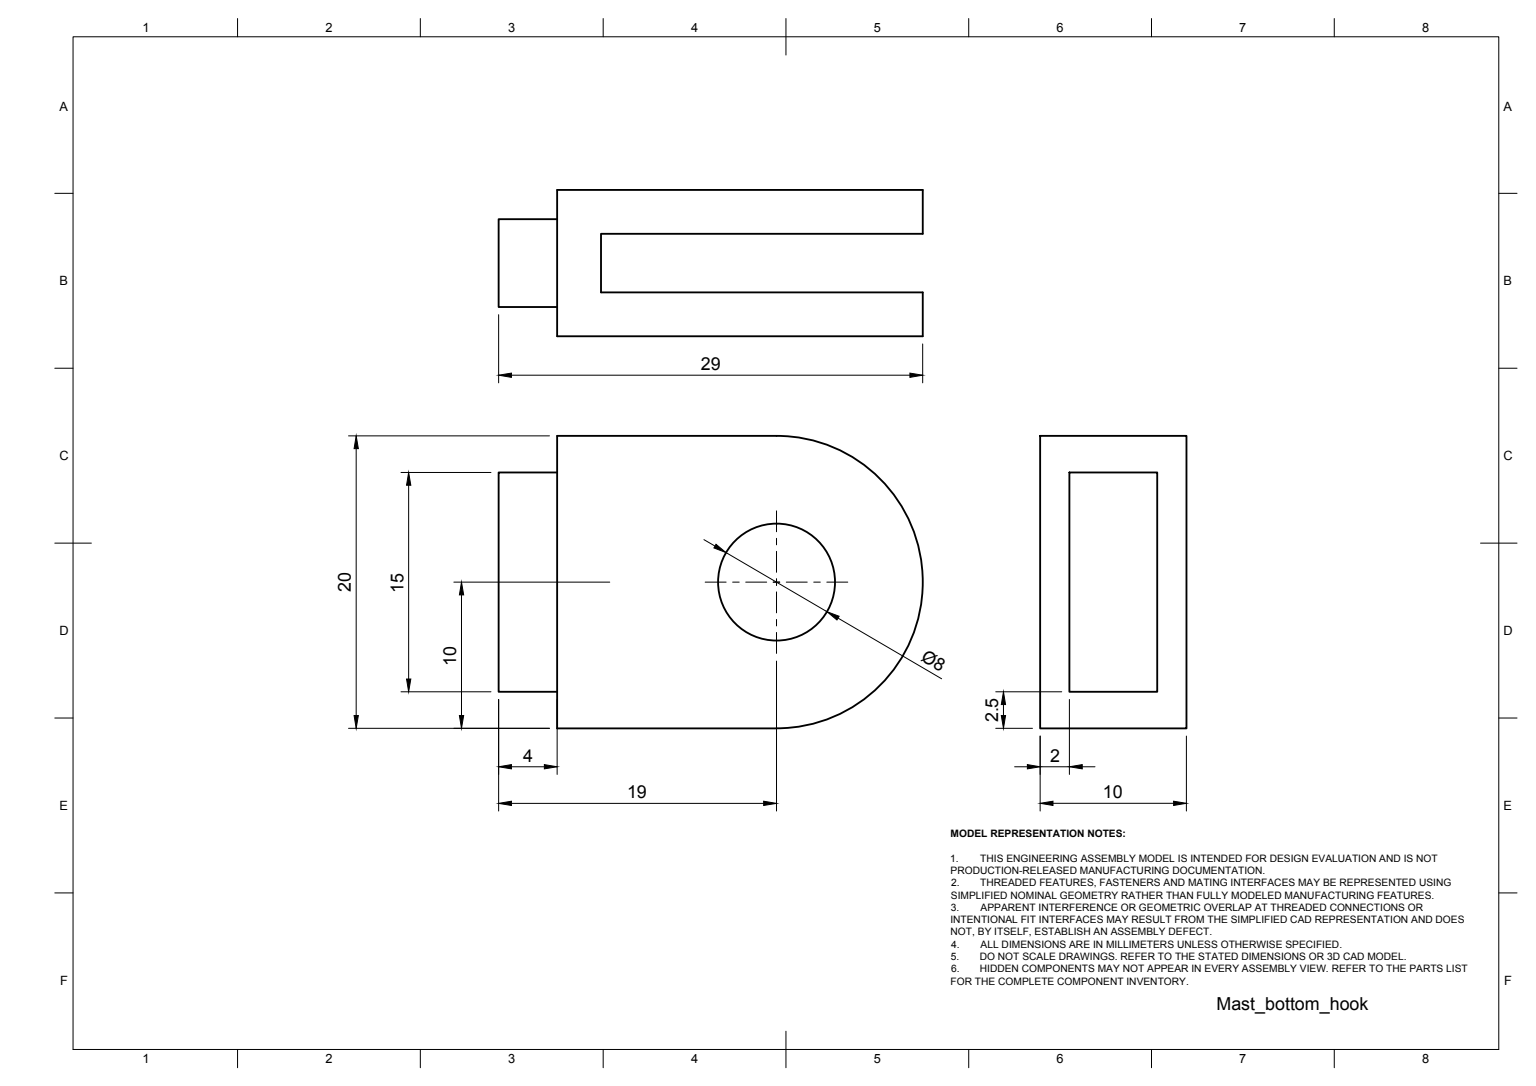
ISO-10303-21;
HEADER;
/* Generated by software containing ST-Developer
 * from STEP Tools, Inc. (www.steptools.com) 
 */

FILE_DESCRIPTION(
/* description */ (''),
/* implementation_level */ '2;1');

FILE_NAME(
/* name */ 'Mast_bottom_hook.step',
/* time_stamp */ '2026-10-07T11:02:43-07:00',
/* author */ (''),
/* organization */ (''),
/* preprocessor_version */ 'ST-DEVELOPER v20.2',
/* originating_system */ 'Autodesk Translation Framework v15.15.0.0',
/* authorisation */ '');

FILE_SCHEMA (('AUTOMOTIVE_DESIGN { 1 0 10303 214 3 1 1 }'));
ENDSEC;

DATA;
#10=MECHANICAL_DESIGN_GEOMETRIC_PRESENTATION_REPRESENTATION('',(#71),#5505);
#57=SHAPE_REPRESENTATION_RELATIONSHIP('SRR','None',#5542,#64);
#64=ADVANCED_BREP_SHAPE_REPRESENTATION('',(#78),#5503);
#71=STYLED_ITEM('',(#5586),#78);
#78=MANIFOLD_SOLID_BREP('Body1',#3298);
#103=FACE_BOUND('',#554,.T.);
#104=FACE_BOUND('',#556,.T.);
#105=FACE_BOUND('',#558,.T.);
#106=FACE_BOUND('',#560,.T.);
#107=FACE_BOUND('',#562,.T.);
#143=CYLINDRICAL_SURFACE('',#3592,4.);
#144=CYLINDRICAL_SURFACE('',#3593,4.);
#145=CYLINDRICAL_SURFACE('',#3594,10.);
#146=CYLINDRICAL_SURFACE('',#3595,10.);
#216=CIRCLE('',#3578,10.);
#217=CIRCLE('',#3579,4.);
#218=CIRCLE('',#3581,10.);
#219=CIRCLE('',#3582,4.);
#220=CIRCLE('',#3584,10.);
#221=CIRCLE('',#3585,4.);
#222=CIRCLE('',#3587,10.);
#223=CIRCLE('',#3588,4.);
#364=FACE_OUTER_BOUND('',#553,.T.);
#365=FACE_OUTER_BOUND('',#555,.T.);
#366=FACE_OUTER_BOUND('',#557,.T.);
#367=FACE_OUTER_BOUND('',#559,.T.);
#368=FACE_OUTER_BOUND('',#561,.T.);
#369=FACE_OUTER_BOUND('',#563,.T.);
#370=FACE_OUTER_BOUND('',#564,.T.);
#371=FACE_OUTER_BOUND('',#565,.T.);
#372=FACE_OUTER_BOUND('',#566,.T.);
#373=FACE_OUTER_BOUND('',#567,.T.);
#374=FACE_OUTER_BOUND('',#568,.T.);
#375=FACE_OUTER_BOUND('',#569,.T.);
#376=FACE_OUTER_BOUND('',#570,.T.);
#377=FACE_OUTER_BOUND('',#571,.T.);
#378=FACE_OUTER_BOUND('',#572,.T.);
#379=FACE_OUTER_BOUND('',#573,.T.);
#380=FACE_OUTER_BOUND('',#574,.T.);
#553=EDGE_LOOP('',(#2810,#2811,#2812,#2813));
#554=EDGE_LOOP('',(#2814,#2815,#2816,#2817));
#555=EDGE_LOOP('',(#2818,#2819,#2820,#2821));
#556=EDGE_LOOP('',(#2822));
#557=EDGE_LOOP('',(#2823,#2824,#2825,#2826));
#558=EDGE_LOOP('',(#2827));
#559=EDGE_LOOP('',(#2828,#2829,#2830,#2831));
#560=EDGE_LOOP('',(#2832));
#561=EDGE_LOOP('',(#2833,#2834,#2835,#2836));
#562=EDGE_LOOP('',(#2837));
#563=EDGE_LOOP('',(#2838,#2839,#2840,#2841,#2842,#2843,#2844,#2845));
#564=EDGE_LOOP('',(#2846,#2847,#2848,#2849,#2850,#2851,#2852,#2853));
#565=EDGE_LOOP('',(#2854,#2855,#2856,#2857));
#566=EDGE_LOOP('',(#2858,#2859,#2860,#2861));
#567=EDGE_LOOP('',(#2862,#2863,#2864,#2865));
#568=EDGE_LOOP('',(#2866,#2867,#2868,#2869));
#569=EDGE_LOOP('',(#2870,#2871,#2872,#2873));
#570=EDGE_LOOP('',(#2874,#2875,#2876,#2877));
#571=EDGE_LOOP('',(#2878,#2879,#2880,#2881));
#572=EDGE_LOOP('',(#2882,#2883,#2884,#2885));
#573=EDGE_LOOP('',(#2886,#2887,#2888,#2889));
#574=EDGE_LOOP('',(#2890,#2891,#2892,#2893));
#895=LINE('',#5282,#1265);
#896=LINE('',#5284,#1266);
#897=LINE('',#5286,#1267);
#898=LINE('',#5287,#1268);
#899=LINE('',#5290,#1269);
#900=LINE('',#5292,#1270);
#901=LINE('',#5294,#1271);
#902=LINE('',#5295,#1272);
#903=LINE('',#5298,#1273);
#904=LINE('',#5301,#1274);
#905=LINE('',#5308,#1275);
#906=LINE('',#5309,#1276);
#907=LINE('',#5315,#1277);
#908=LINE('',#5319,#1278);
#909=LINE('',#5320,#1279);
#910=LINE('',#5326,#1280);
#911=LINE('',#5330,#1281);
#912=LINE('',#5331,#1282);
#913=LINE('',#5335,#1283);
#914=LINE('',#5336,#1284);
#915=LINE('',#5337,#1285);
#916=LINE('',#5339,#1286);
#917=LINE('',#5340,#1287);
#918=LINE('',#5341,#1288);
#919=LINE('',#5344,#1289);
#920=LINE('',#5346,#1290);
#921=LINE('',#5351,#1291);
#922=LINE('',#5353,#1292);
#923=LINE('',#5354,#1293);
#924=LINE('',#5357,#1294);
#925=LINE('',#5358,#1295);
#926=LINE('',#5361,#1296);
#927=LINE('',#5362,#1297);
#928=LINE('',#5364,#1298);
#1265=VECTOR('',#4337,1000.);
#1266=VECTOR('',#4338,1000.);
#1267=VECTOR('',#4339,1000.);
#1268=VECTOR('',#4340,1000.);
#1269=VECTOR('',#4341,1000.);
#1270=VECTOR('',#4342,1000.);
#1271=VECTOR('',#4343,1000.);
#1272=VECTOR('',#4344,1000.);
#1273=VECTOR('',#4347,1000.);
#1274=VECTOR('',#4350,1000.);
#1275=VECTOR('',#4357,1000.);
#1276=VECTOR('',#4358,1000.);
#1277=VECTOR('',#4363,1000.);
#1278=VECTOR('',#4366,1000.);
#1279=VECTOR('',#4367,1000.);
#1280=VECTOR('',#4372,1000.);
#1281=VECTOR('',#4375,1000.);
#1282=VECTOR('',#4376,1000.);
#1283=VECTOR('',#4381,1000.);
#1284=VECTOR('',#4382,1000.);
#1285=VECTOR('',#4383,1000.);
#1286=VECTOR('',#4386,1000.);
#1287=VECTOR('',#4387,1000.);
#1288=VECTOR('',#4388,1000.);
#1289=VECTOR('',#4393,4.);
#1290=VECTOR('',#4396,4.);
#1291=VECTOR('',#4403,1000.);
#1292=VECTOR('',#4404,1000.);
#1293=VECTOR('',#4405,1000.);
#1294=VECTOR('',#4408,1000.);
#1295=VECTOR('',#4409,1000.);
#1296=VECTOR('',#4412,1000.);
#1297=VECTOR('',#4413,1000.);
#1298=VECTOR('',#4416,1000.);
#1579=VERTEX_POINT('',#5280);
#1580=VERTEX_POINT('',#5281);
#1581=VERTEX_POINT('',#5283);
#1582=VERTEX_POINT('',#5285);
#1583=VERTEX_POINT('',#5288);
#1584=VERTEX_POINT('',#5289);
#1585=VERTEX_POINT('',#5291);
#1586=VERTEX_POINT('',#5293);
#1587=VERTEX_POINT('',#5297);
#1588=VERTEX_POINT('',#5299);
#1589=VERTEX_POINT('',#5302);
#1590=VERTEX_POINT('',#5305);
#1591=VERTEX_POINT('',#5306);
#1592=VERTEX_POINT('',#5310);
#1593=VERTEX_POINT('',#5313);
#1594=VERTEX_POINT('',#5314);
#1595=VERTEX_POINT('',#5316);
#1596=VERTEX_POINT('',#5318);
#1597=VERTEX_POINT('',#5321);
#1598=VERTEX_POINT('',#5324);
#1599=VERTEX_POINT('',#5325);
#1600=VERTEX_POINT('',#5327);
#1601=VERTEX_POINT('',#5329);
#1602=VERTEX_POINT('',#5332);
#1603=VERTEX_POINT('',#5350);
#1604=VERTEX_POINT('',#5352);
#1605=VERTEX_POINT('',#5356);
#1606=VERTEX_POINT('',#5360);
#2000=EDGE_CURVE('',#1579,#1580,#895,.T.);
#2001=EDGE_CURVE('',#1581,#1580,#896,.T.);
#2002=EDGE_CURVE('',#1582,#1581,#897,.T.);
#2003=EDGE_CURVE('',#1582,#1579,#898,.T.);
#2004=EDGE_CURVE('',#1583,#1584,#899,.T.);
#2005=EDGE_CURVE('',#1583,#1585,#900,.T.);
#2006=EDGE_CURVE('',#1585,#1586,#901,.T.);
#2007=EDGE_CURVE('',#1584,#1586,#902,.T.);
#2008=EDGE_CURVE('',#1587,#1579,#903,.T.);
#2009=EDGE_CURVE('',#1587,#1588,#216,.T.);
#2010=EDGE_CURVE('',#1588,#1580,#904,.T.);
#2011=EDGE_CURVE('',#1589,#1589,#217,.T.);
#2012=EDGE_CURVE('',#1590,#1591,#218,.T.);
#2013=EDGE_CURVE('',#1590,#1582,#905,.T.);
#2014=EDGE_CURVE('',#1591,#1581,#906,.T.);
#2015=EDGE_CURVE('',#1592,#1592,#219,.T.);
#2016=EDGE_CURVE('',#1593,#1594,#907,.T.);
#2017=EDGE_CURVE('',#1594,#1595,#220,.T.);
#2018=EDGE_CURVE('',#1596,#1595,#908,.T.);
#2019=EDGE_CURVE('',#1596,#1593,#909,.T.);
#2020=EDGE_CURVE('',#1597,#1597,#221,.T.);
#2021=EDGE_CURVE('',#1598,#1599,#910,.T.);
#2022=EDGE_CURVE('',#1600,#1599,#222,.T.);
#2023=EDGE_CURVE('',#1601,#1600,#911,.T.);
#2024=EDGE_CURVE('',#1598,#1601,#912,.T.);
#2025=EDGE_CURVE('',#1602,#1602,#223,.T.);
#2026=EDGE_CURVE('',#1595,#1587,#913,.T.);
#2027=EDGE_CURVE('',#1590,#1599,#914,.T.);
#2028=EDGE_CURVE('',#1598,#1596,#915,.T.);
#2029=EDGE_CURVE('',#1594,#1588,#916,.T.);
#2030=EDGE_CURVE('',#1601,#1593,#917,.T.);
#2031=EDGE_CURVE('',#1591,#1600,#918,.T.);
#2032=EDGE_CURVE('',#1592,#1602,#919,.T.);
#2033=EDGE_CURVE('',#1597,#1589,#920,.T.);
#2034=EDGE_CURVE('',#1603,#1584,#921,.T.);
#2035=EDGE_CURVE('',#1604,#1603,#922,.T.);
#2036=EDGE_CURVE('',#1604,#1583,#923,.T.);
#2037=EDGE_CURVE('',#1604,#1605,#924,.T.);
#2038=EDGE_CURVE('',#1605,#1585,#925,.T.);
#2039=EDGE_CURVE('',#1605,#1606,#926,.T.);
#2040=EDGE_CURVE('',#1606,#1586,#927,.T.);
#2041=EDGE_CURVE('',#1603,#1606,#928,.T.);
#2810=ORIENTED_EDGE('',*,*,#2000,.T.);
#2811=ORIENTED_EDGE('',*,*,#2001,.F.);
#2812=ORIENTED_EDGE('',*,*,#2002,.F.);
#2813=ORIENTED_EDGE('',*,*,#2003,.T.);
#2814=ORIENTED_EDGE('',*,*,#2004,.F.);
#2815=ORIENTED_EDGE('',*,*,#2005,.T.);
#2816=ORIENTED_EDGE('',*,*,#2006,.T.);
#2817=ORIENTED_EDGE('',*,*,#2007,.F.);
#2818=ORIENTED_EDGE('',*,*,#2008,.F.);
#2819=ORIENTED_EDGE('',*,*,#2009,.T.);
#2820=ORIENTED_EDGE('',*,*,#2010,.T.);
#2821=ORIENTED_EDGE('',*,*,#2000,.F.);
#2822=ORIENTED_EDGE('',*,*,#2011,.F.);
#2823=ORIENTED_EDGE('',*,*,#2012,.F.);
#2824=ORIENTED_EDGE('',*,*,#2013,.T.);
#2825=ORIENTED_EDGE('',*,*,#2002,.T.);
#2826=ORIENTED_EDGE('',*,*,#2014,.F.);
#2827=ORIENTED_EDGE('',*,*,#2015,.T.);
#2828=ORIENTED_EDGE('',*,*,#2016,.T.);
#2829=ORIENTED_EDGE('',*,*,#2017,.T.);
#2830=ORIENTED_EDGE('',*,*,#2018,.F.);
#2831=ORIENTED_EDGE('',*,*,#2019,.T.);
#2832=ORIENTED_EDGE('',*,*,#2020,.F.);
#2833=ORIENTED_EDGE('',*,*,#2021,.T.);
#2834=ORIENTED_EDGE('',*,*,#2022,.F.);
#2835=ORIENTED_EDGE('',*,*,#2023,.F.);
#2836=ORIENTED_EDGE('',*,*,#2024,.F.);
#2837=ORIENTED_EDGE('',*,*,#2025,.T.);
#2838=ORIENTED_EDGE('',*,*,#2026,.T.);
#2839=ORIENTED_EDGE('',*,*,#2008,.T.);
#2840=ORIENTED_EDGE('',*,*,#2003,.F.);
#2841=ORIENTED_EDGE('',*,*,#2013,.F.);
#2842=ORIENTED_EDGE('',*,*,#2027,.T.);
#2843=ORIENTED_EDGE('',*,*,#2021,.F.);
#2844=ORIENTED_EDGE('',*,*,#2028,.T.);
#2845=ORIENTED_EDGE('',*,*,#2018,.T.);
#2846=ORIENTED_EDGE('',*,*,#2010,.F.);
#2847=ORIENTED_EDGE('',*,*,#2029,.F.);
#2848=ORIENTED_EDGE('',*,*,#2016,.F.);
#2849=ORIENTED_EDGE('',*,*,#2030,.F.);
#2850=ORIENTED_EDGE('',*,*,#2023,.T.);
#2851=ORIENTED_EDGE('',*,*,#2031,.F.);
#2852=ORIENTED_EDGE('',*,*,#2014,.T.);
#2853=ORIENTED_EDGE('',*,*,#2001,.T.);
#2854=ORIENTED_EDGE('',*,*,#2024,.T.);
#2855=ORIENTED_EDGE('',*,*,#2030,.T.);
#2856=ORIENTED_EDGE('',*,*,#2019,.F.);
#2857=ORIENTED_EDGE('',*,*,#2028,.F.);
#2858=ORIENTED_EDGE('',*,*,#2015,.F.);
#2859=ORIENTED_EDGE('',*,*,#2032,.T.);
#2860=ORIENTED_EDGE('',*,*,#2025,.F.);
#2861=ORIENTED_EDGE('',*,*,#2032,.F.);
#2862=ORIENTED_EDGE('',*,*,#2020,.T.);
#2863=ORIENTED_EDGE('',*,*,#2033,.T.);
#2864=ORIENTED_EDGE('',*,*,#2011,.T.);
#2865=ORIENTED_EDGE('',*,*,#2033,.F.);
#2866=ORIENTED_EDGE('',*,*,#2012,.T.);
#2867=ORIENTED_EDGE('',*,*,#2031,.T.);
#2868=ORIENTED_EDGE('',*,*,#2022,.T.);
#2869=ORIENTED_EDGE('',*,*,#2027,.F.);
#2870=ORIENTED_EDGE('',*,*,#2017,.F.);
#2871=ORIENTED_EDGE('',*,*,#2029,.T.);
#2872=ORIENTED_EDGE('',*,*,#2009,.F.);
#2873=ORIENTED_EDGE('',*,*,#2026,.F.);
#2874=ORIENTED_EDGE('',*,*,#2004,.T.);
#2875=ORIENTED_EDGE('',*,*,#2034,.F.);
#2876=ORIENTED_EDGE('',*,*,#2035,.F.);
#2877=ORIENTED_EDGE('',*,*,#2036,.T.);
#2878=ORIENTED_EDGE('',*,*,#2005,.F.);
#2879=ORIENTED_EDGE('',*,*,#2036,.F.);
#2880=ORIENTED_EDGE('',*,*,#2037,.T.);
#2881=ORIENTED_EDGE('',*,*,#2038,.T.);
#2882=ORIENTED_EDGE('',*,*,#2006,.F.);
#2883=ORIENTED_EDGE('',*,*,#2038,.F.);
#2884=ORIENTED_EDGE('',*,*,#2039,.T.);
#2885=ORIENTED_EDGE('',*,*,#2040,.T.);
#2886=ORIENTED_EDGE('',*,*,#2007,.T.);
#2887=ORIENTED_EDGE('',*,*,#2040,.F.);
#2888=ORIENTED_EDGE('',*,*,#2041,.F.);
#2889=ORIENTED_EDGE('',*,*,#2034,.T.);
#2890=ORIENTED_EDGE('',*,*,#2035,.T.);
#2891=ORIENTED_EDGE('',*,*,#2041,.T.);
#2892=ORIENTED_EDGE('',*,*,#2039,.F.);
#2893=ORIENTED_EDGE('',*,*,#2037,.F.);
#3099=PLANE('',#3576);
#3100=PLANE('',#3577);
#3101=PLANE('',#3580);
#3102=PLANE('',#3583);
#3103=PLANE('',#3586);
#3104=PLANE('',#3589);
#3105=PLANE('',#3590);
#3106=PLANE('',#3591);
#3107=PLANE('',#3596);
#3108=PLANE('',#3597);
#3109=PLANE('',#3598);
#3110=PLANE('',#3599);
#3111=PLANE('',#3600);
#3255=ADVANCED_FACE('',(#364,#103),#3099,.F.);
#3256=ADVANCED_FACE('',(#365,#104),#3100,.T.);
#3257=ADVANCED_FACE('',(#366,#105),#3101,.F.);
#3258=ADVANCED_FACE('',(#367,#106),#3102,.T.);
#3259=ADVANCED_FACE('',(#368,#107),#3103,.F.);
#3260=ADVANCED_FACE('',(#369),#3104,.T.);
#3261=ADVANCED_FACE('',(#370),#3105,.F.);
#3262=ADVANCED_FACE('',(#371),#3106,.T.);
#3263=ADVANCED_FACE('',(#372),#143,.F.);
#3264=ADVANCED_FACE('',(#373),#144,.F.);
#3265=ADVANCED_FACE('',(#374),#145,.T.);
#3266=ADVANCED_FACE('',(#375),#146,.T.);
#3267=ADVANCED_FACE('',(#376),#3107,.F.);
#3268=ADVANCED_FACE('',(#377),#3108,.T.);
#3269=ADVANCED_FACE('',(#378),#3109,.T.);
#3270=ADVANCED_FACE('',(#379),#3110,.F.);
#3271=ADVANCED_FACE('',(#380),#3111,.F.);
#3298=CLOSED_SHELL('',(#3255,#3256,#3257,#3258,#3259,#3260,#3261,#3262,
#3263,#3264,#3265,#3266,#3267,#3268,#3269,#3270,#3271));
#3575=AXIS2_PLACEMENT_3D('',#5278,#4333,#4334);
#3576=AXIS2_PLACEMENT_3D('',#5279,#4335,#4336);
#3577=AXIS2_PLACEMENT_3D('',#5296,#4345,#4346);
#3578=AXIS2_PLACEMENT_3D('',#5300,#4348,#4349);
#3579=AXIS2_PLACEMENT_3D('',#5303,#4351,#4352);
#3580=AXIS2_PLACEMENT_3D('',#5304,#4353,#4354);
#3581=AXIS2_PLACEMENT_3D('',#5307,#4355,#4356);
#3582=AXIS2_PLACEMENT_3D('',#5311,#4359,#4360);
#3583=AXIS2_PLACEMENT_3D('',#5312,#4361,#4362);
#3584=AXIS2_PLACEMENT_3D('',#5317,#4364,#4365);
#3585=AXIS2_PLACEMENT_3D('',#5322,#4368,#4369);
#3586=AXIS2_PLACEMENT_3D('',#5323,#4370,#4371);
#3587=AXIS2_PLACEMENT_3D('',#5328,#4373,#4374);
#3588=AXIS2_PLACEMENT_3D('',#5333,#4377,#4378);
#3589=AXIS2_PLACEMENT_3D('',#5334,#4379,#4380);
#3590=AXIS2_PLACEMENT_3D('',#5338,#4384,#4385);
#3591=AXIS2_PLACEMENT_3D('',#5342,#4389,#4390);
#3592=AXIS2_PLACEMENT_3D('',#5343,#4391,#4392);
#3593=AXIS2_PLACEMENT_3D('',#5345,#4394,#4395);
#3594=AXIS2_PLACEMENT_3D('',#5347,#4397,#4398);
#3595=AXIS2_PLACEMENT_3D('',#5348,#4399,#4400);
#3596=AXIS2_PLACEMENT_3D('',#5349,#4401,#4402);
#3597=AXIS2_PLACEMENT_3D('',#5355,#4406,#4407);
#3598=AXIS2_PLACEMENT_3D('',#5359,#4410,#4411);
#3599=AXIS2_PLACEMENT_3D('',#5363,#4414,#4415);
#3600=AXIS2_PLACEMENT_3D('',#5365,#4417,#4418);
#4333=DIRECTION('axis',(0.,0.,1.));
#4334=DIRECTION('refdir',(1.,0.,0.));
#4335=DIRECTION('center_axis',(3.06161699786839E-16,-5.78241158658936E-16,
1.));
#4336=DIRECTION('ref_axis',(1.,1.77035296021731E-31,-3.06161699786839E-16));
#4337=DIRECTION('',(-1.77035296021731E-31,-1.,-5.78241158658936E-16));
#4338=DIRECTION('',(1.,1.77035296021731E-31,-3.06161699786839E-16));
#4339=DIRECTION('',(-1.77035296021731E-31,-1.,-5.78241158658936E-16));
#4340=DIRECTION('',(1.,1.77035296021731E-31,-3.06161699786839E-16));
#4341=DIRECTION('',(1.77035296021731E-31,1.,5.78241158658936E-16));
#4342=DIRECTION('',(1.,1.77035296021731E-31,-3.06161699786839E-16));
#4343=DIRECTION('',(1.77035296021731E-31,1.,5.78241158658936E-16));
#4344=DIRECTION('',(1.,1.77035296021731E-31,-3.06161699786839E-16));
#4345=DIRECTION('center_axis',(1.,-2.73691106313441E-47,-3.06161699786839E-16));
#4346=DIRECTION('ref_axis',(-3.06161699786839E-16,0.,-1.));
#4347=DIRECTION('',(-3.06161699786839E-16,5.78241158658936E-16,-1.));
#4348=DIRECTION('center_axis',(1.,-2.73691106313441E-47,-3.06161699786839E-16));
#4349=DIRECTION('ref_axis',(-3.06161699786839E-16,0.,-1.));
#4350=DIRECTION('',(-3.06161699786839E-16,5.78241158658936E-16,-1.));
#4351=DIRECTION('center_axis',(1.,-2.73691106313441E-47,-3.06161699786839E-16));
#4352=DIRECTION('ref_axis',(-3.06161699786839E-16,0.,-1.));
#4353=DIRECTION('center_axis',(1.,-2.73691106313441E-47,-3.06161699786839E-16));
#4354=DIRECTION('ref_axis',(-3.06161699786839E-16,0.,-1.));
#4355=DIRECTION('center_axis',(1.,-2.73691106313441E-47,-3.06161699786839E-16));
#4356=DIRECTION('ref_axis',(-3.06161699786839E-16,0.,-1.));
#4357=DIRECTION('',(-3.06161699786839E-16,5.78241158658936E-16,-1.));
#4358=DIRECTION('',(-3.06161699786839E-16,5.78241158658936E-16,-1.));
#4359=DIRECTION('center_axis',(1.,-2.73691106313441E-47,-3.06161699786839E-16));
#4360=DIRECTION('ref_axis',(-3.06161699786839E-16,0.,-1.));
#4361=DIRECTION('center_axis',(-1.,0.,3.06161699786839E-16));
#4362=DIRECTION('ref_axis',(3.06161699786839E-16,0.,1.));
#4363=DIRECTION('',(3.06161699786839E-16,-5.78241158658936E-16,1.));
#4364=DIRECTION('center_axis',(-1.,0.,3.06161699786839E-16));
#4365=DIRECTION('ref_axis',(3.06161699786839E-16,0.,1.));
#4366=DIRECTION('',(3.06161699786839E-16,-5.78241158658936E-16,1.));
#4367=DIRECTION('',(-1.77035296021731E-31,-1.,-5.78241158658936E-16));
#4368=DIRECTION('center_axis',(-1.,0.,3.06161699786839E-16));
#4369=DIRECTION('ref_axis',(3.06161699786839E-16,0.,1.));
#4370=DIRECTION('center_axis',(-1.,0.,3.06161699786839E-16));
#4371=DIRECTION('ref_axis',(3.06161699786839E-16,0.,1.));
#4372=DIRECTION('',(3.06161699786839E-16,-5.78241158658936E-16,1.));
#4373=DIRECTION('center_axis',(-1.,0.,3.06161699786839E-16));
#4374=DIRECTION('ref_axis',(3.06161699786839E-16,0.,1.));
#4375=DIRECTION('',(3.06161699786839E-16,-5.78241158658936E-16,1.));
#4376=DIRECTION('',(-1.77035296021731E-31,-1.,-5.78241158658936E-16));
#4377=DIRECTION('center_axis',(-1.,0.,3.06161699786839E-16));
#4378=DIRECTION('ref_axis',(3.06161699786839E-16,0.,1.));
#4379=DIRECTION('center_axis',(0.,1.,5.78241158658936E-16));
#4380=DIRECTION('ref_axis',(0.,-5.78241158658936E-16,1.));
#4381=DIRECTION('',(1.,-2.73691106313441E-47,-3.06161699786839E-16));
#4382=DIRECTION('',(1.,-2.73691106313441E-47,-3.06161699786839E-16));
#4383=DIRECTION('',(1.,1.77035296021731E-31,-3.06161699786839E-16));
#4384=DIRECTION('center_axis',(0.,1.,5.78241158658936E-16));
#4385=DIRECTION('ref_axis',(0.,-5.78241158658936E-16,1.));
#4386=DIRECTION('',(1.,-2.73691106313441E-47,-3.06161699786839E-16));
#4387=DIRECTION('',(1.,1.77035296021731E-31,-3.06161699786839E-16));
#4388=DIRECTION('',(1.,-2.73691106313441E-47,-3.06161699786839E-16));
#4389=DIRECTION('center_axis',(3.06161699786839E-16,-5.78241158658936E-16,
1.));
#4390=DIRECTION('ref_axis',(1.,1.77035296021731E-31,-3.06161699786839E-16));
#4391=DIRECTION('center_axis',(1.,-2.73691106313441E-47,-3.06161699786839E-16));
#4392=DIRECTION('ref_axis',(-3.06161699786839E-16,0.,-1.));
#4393=DIRECTION('',(1.,-2.73691106313441E-47,-3.06161699786839E-16));
#4394=DIRECTION('center_axis',(1.,-2.73691106313441E-47,-3.06161699786839E-16));
#4395=DIRECTION('ref_axis',(-3.06161699786839E-16,0.,-1.));
#4396=DIRECTION('',(1.,-2.73691106313441E-47,-3.06161699786839E-16));
#4397=DIRECTION('center_axis',(1.,-2.73691106313441E-47,-3.06161699786839E-16));
#4398=DIRECTION('ref_axis',(3.06161699786839E-16,1.22464679914735E-16,1.));
#4399=DIRECTION('center_axis',(1.,-2.73691106313441E-47,-3.06161699786839E-16));
#4400=DIRECTION('ref_axis',(3.06161699786839E-16,1.22464679914735E-16,1.));
#4401=DIRECTION('center_axis',(1.,-2.13821176807375E-47,-3.06161699786839E-16));
#4402=DIRECTION('ref_axis',(-3.06161699786839E-16,0.,-1.));
#4403=DIRECTION('',(3.06161699786839E-16,-5.78241158658936E-16,1.));
#4404=DIRECTION('',(1.77035296021731E-31,1.,5.78241158658936E-16));
#4405=DIRECTION('',(3.06161699786839E-16,-5.78241158658936E-16,1.));
#4406=DIRECTION('center_axis',(2.13821176807375E-47,-1.,-5.78241158658936E-16));
#4407=DIRECTION('ref_axis',(-7.75905768621749E-79,5.78241158658936E-16,
-1.));
#4408=DIRECTION('',(1.,1.77035296021731E-31,-3.06161699786839E-16));
#4409=DIRECTION('',(3.06161699786839E-16,-5.78241158658936E-16,1.));
#4410=DIRECTION('center_axis',(1.,-2.13821176807375E-47,-3.06161699786839E-16));
#4411=DIRECTION('ref_axis',(-3.06161699786839E-16,0.,-1.));
#4412=DIRECTION('',(1.77035296021731E-31,1.,5.78241158658936E-16));
#4413=DIRECTION('',(3.06161699786839E-16,-5.78241158658936E-16,1.));
#4414=DIRECTION('center_axis',(2.13821176807375E-47,-1.,-5.78241158658936E-16));
#4415=DIRECTION('ref_axis',(-7.75905768621749E-79,5.78241158658936E-16,
-1.));
#4416=DIRECTION('',(1.,1.77035296021731E-31,-3.06161699786839E-16));
#4417=DIRECTION('center_axis',(3.06161699786839E-16,-5.78241158658936E-16,
1.));
#4418=DIRECTION('ref_axis',(1.,1.77035296021731E-31,-3.06161699786839E-16));
#5278=CARTESIAN_POINT('',(0.,0.,0.));
#5279=CARTESIAN_POINT('Origin',(5.2659812363336E-14,876.65182352066,172.));
#5280=CARTESIAN_POINT('',(-150.,860.,172.));
#5281=CARTESIAN_POINT('',(-150.,840.,172.));
#5282=CARTESIAN_POINT('',(-150.,850.,172.));
#5283=CARTESIAN_POINT('',(-160.,840.,172.));
#5284=CARTESIAN_POINT('',(-155.,840.,172.));
#5285=CARTESIAN_POINT('',(-160.,860.,172.));
#5286=CARTESIAN_POINT('',(-160.,850.,172.));
#5287=CARTESIAN_POINT('',(-155.,860.,172.));
#5288=CARTESIAN_POINT('',(-158.,842.5,172.));
#5289=CARTESIAN_POINT('',(-158.,857.5,172.));
#5290=CARTESIAN_POINT('',(-158.,850.,172.));
#5291=CARTESIAN_POINT('',(-152.,842.5,172.));
#5292=CARTESIAN_POINT('',(-155.,842.5,172.));
#5293=CARTESIAN_POINT('',(-152.,857.5,172.));
#5294=CARTESIAN_POINT('',(-152.,850.,172.));
#5295=CARTESIAN_POINT('',(-155.,857.5,172.));
#5296=CARTESIAN_POINT('Origin',(-150.,850.,197.));
#5297=CARTESIAN_POINT('',(-150.,860.,187.));
#5298=CARTESIAN_POINT('',(-150.,860.,197.));
#5299=CARTESIAN_POINT('',(-150.,840.,187.));
#5300=CARTESIAN_POINT('Origin',(-150.,850.,187.));
#5301=CARTESIAN_POINT('',(-150.,840.,197.));
#5302=CARTESIAN_POINT('',(-150.,850.,190.999999999999));
#5303=CARTESIAN_POINT('Origin',(-150.,850.,187.));
#5304=CARTESIAN_POINT('Origin',(-160.,850.,197.));
#5305=CARTESIAN_POINT('',(-160.,860.,187.));
#5306=CARTESIAN_POINT('',(-160.,840.,187.));
#5307=CARTESIAN_POINT('Origin',(-160.,850.,187.));
#5308=CARTESIAN_POINT('',(-160.,860.,197.));
#5309=CARTESIAN_POINT('',(-160.,840.,197.));
#5310=CARTESIAN_POINT('',(-160.,850.,190.999999999999));
#5311=CARTESIAN_POINT('Origin',(-160.,850.,187.));
#5312=CARTESIAN_POINT('Origin',(-153.,850.,175.));
#5313=CARTESIAN_POINT('',(-153.,840.,175.));
#5314=CARTESIAN_POINT('',(-153.,840.,187.));
#5315=CARTESIAN_POINT('',(-153.,840.,197.));
#5316=CARTESIAN_POINT('',(-153.,860.,187.));
#5317=CARTESIAN_POINT('Origin',(-153.,850.,187.));
#5318=CARTESIAN_POINT('',(-153.,860.,175.));
#5319=CARTESIAN_POINT('',(-153.,860.,197.));
#5320=CARTESIAN_POINT('',(-153.,850.,175.));
#5321=CARTESIAN_POINT('',(-153.,850.,191.));
#5322=CARTESIAN_POINT('Origin',(-153.,850.,187.));
#5323=CARTESIAN_POINT('Origin',(-157.,850.,175.));
#5324=CARTESIAN_POINT('',(-157.,860.,175.));
#5325=CARTESIAN_POINT('',(-157.,860.,187.));
#5326=CARTESIAN_POINT('',(-157.,860.,197.));
#5327=CARTESIAN_POINT('',(-157.,840.,187.));
#5328=CARTESIAN_POINT('Origin',(-157.,850.,187.));
#5329=CARTESIAN_POINT('',(-157.,840.,175.));
#5330=CARTESIAN_POINT('',(-157.,840.,197.));
#5331=CARTESIAN_POINT('',(-157.,850.,175.));
#5332=CARTESIAN_POINT('',(-157.,850.,191.));
#5333=CARTESIAN_POINT('Origin',(-157.,850.,187.));
#5334=CARTESIAN_POINT('Origin',(-155.,860.,197.));
#5335=CARTESIAN_POINT('',(-3269.52807175403,860.,187.));
#5336=CARTESIAN_POINT('',(-3269.52807175403,860.,187.));
#5337=CARTESIAN_POINT('',(-155.,860.,175.));
#5338=CARTESIAN_POINT('Origin',(-155.,840.,197.));
#5339=CARTESIAN_POINT('',(-3269.52807175403,840.,187.));
#5340=CARTESIAN_POINT('',(-155.,840.,175.));
#5341=CARTESIAN_POINT('',(-3269.52807175403,840.,187.));
#5342=CARTESIAN_POINT('Origin',(-155.,850.,175.));
#5343=CARTESIAN_POINT('Origin',(-3269.52807175403,850.,187.));
#5344=CARTESIAN_POINT('',(-3269.52807175403,850.,191.));
#5345=CARTESIAN_POINT('Origin',(-3269.52807175403,850.,187.));
#5346=CARTESIAN_POINT('',(-3269.52807175403,850.,191.));
#5347=CARTESIAN_POINT('Origin',(-3269.52807175403,850.,187.));
#5348=CARTESIAN_POINT('Origin',(-3269.52807175403,850.,187.));
#5349=CARTESIAN_POINT('Origin',(-158.,850.,168.));
#5350=CARTESIAN_POINT('',(-158.,857.5,168.));
#5351=CARTESIAN_POINT('',(-158.,857.5,168.));
#5352=CARTESIAN_POINT('',(-158.,842.5,168.));
#5353=CARTESIAN_POINT('',(-158.,850.,168.));
#5354=CARTESIAN_POINT('',(-158.,842.5,168.));
#5355=CARTESIAN_POINT('Origin',(-155.,842.5,168.));
#5356=CARTESIAN_POINT('',(-152.,842.5,168.));
#5357=CARTESIAN_POINT('',(-155.,842.5,168.));
#5358=CARTESIAN_POINT('',(-152.,842.5,168.));
#5359=CARTESIAN_POINT('Origin',(-152.,850.,168.));
#5360=CARTESIAN_POINT('',(-152.,857.5,168.));
#5361=CARTESIAN_POINT('',(-152.,850.,168.));
#5362=CARTESIAN_POINT('',(-152.,857.5,168.));
#5363=CARTESIAN_POINT('Origin',(-155.,857.5,168.));
#5364=CARTESIAN_POINT('',(-155.,857.5,168.));
#5365=CARTESIAN_POINT('Origin',(-155.,850.,168.));
#5494=UNCERTAINTY_MEASURE_WITH_UNIT(LENGTH_MEASURE(0.01),#5506,
'DISTANCE_ACCURACY_VALUE',
'Maximum model space distance between geometric entities at asserted c
onnectivities');
#5496=UNCERTAINTY_MEASURE_WITH_UNIT(LENGTH_MEASURE(0.01),#5506,
'DISTANCE_ACCURACY_VALUE',
'Maximum model space distance between geometric entities at asserted c
onnectivities');
#5503=(
GEOMETRIC_REPRESENTATION_CONTEXT(3)
GLOBAL_UNCERTAINTY_ASSIGNED_CONTEXT((#5494))
GLOBAL_UNIT_ASSIGNED_CONTEXT((#5506,#5508,#5509))
REPRESENTATION_CONTEXT('','3D')
);
#5505=(
GEOMETRIC_REPRESENTATION_CONTEXT(3)
GLOBAL_UNCERTAINTY_ASSIGNED_CONTEXT((#5496))
GLOBAL_UNIT_ASSIGNED_CONTEXT((#5506,#5508,#5509))
REPRESENTATION_CONTEXT('','3D')
);
#5506=(
LENGTH_UNIT()
NAMED_UNIT(*)
SI_UNIT(.MILLI.,.METRE.)
);
#5508=(
NAMED_UNIT(*)
PLANE_ANGLE_UNIT()
SI_UNIT($,.RADIAN.)
);
#5509=(
NAMED_UNIT(*)
SI_UNIT($,.STERADIAN.)
SOLID_ANGLE_UNIT()
);
#5516=SHAPE_DEFINITION_REPRESENTATION(#5524,#5542);
#5524=PRODUCT_DEFINITION_SHAPE('',$,#5551);
#5542=SHAPE_REPRESENTATION('',(#3575),#5503);
#5544=PRODUCT_DEFINITION_CONTEXT('part definition',#5570,'design');
#5551=PRODUCT_DEFINITION('Mast_bottom_hook','Mast_bottom_hook',#5559,#5544);
#5559=PRODUCT_DEFINITION_FORMATION('',$,#5578);
#5570=APPLICATION_CONTEXT(
'Core Data for Automotive Mechanical Design Process');
#5571=PRODUCT_CONTEXT('part definition',#5570,'mechanical');
#5578=PRODUCT('Mast_bottom_hook','Mast_bottom_hook',
'3mm_8pcs_second_mast_bottom_hook',(#5571));
#5586=PRESENTATION_STYLE_ASSIGNMENT((#5594));
#5594=SURFACE_STYLE_USAGE(.BOTH.,#5602);
#5602=SURFACE_SIDE_STYLE('',(#5610));
#5610=SURFACE_STYLE_FILL_AREA(#5618);
#5618=FILL_AREA_STYLE('Opaque(250,182,1)',(#5626));
#5626=FILL_AREA_STYLE_COLOUR('Opaque(250,182,1)',#5634);
#5634=COLOUR_RGB('Opaque(250,182,1)', 0.08235294, 0.09019608, 0.10196078);
ENDSEC;
END-ISO-10303-21;
